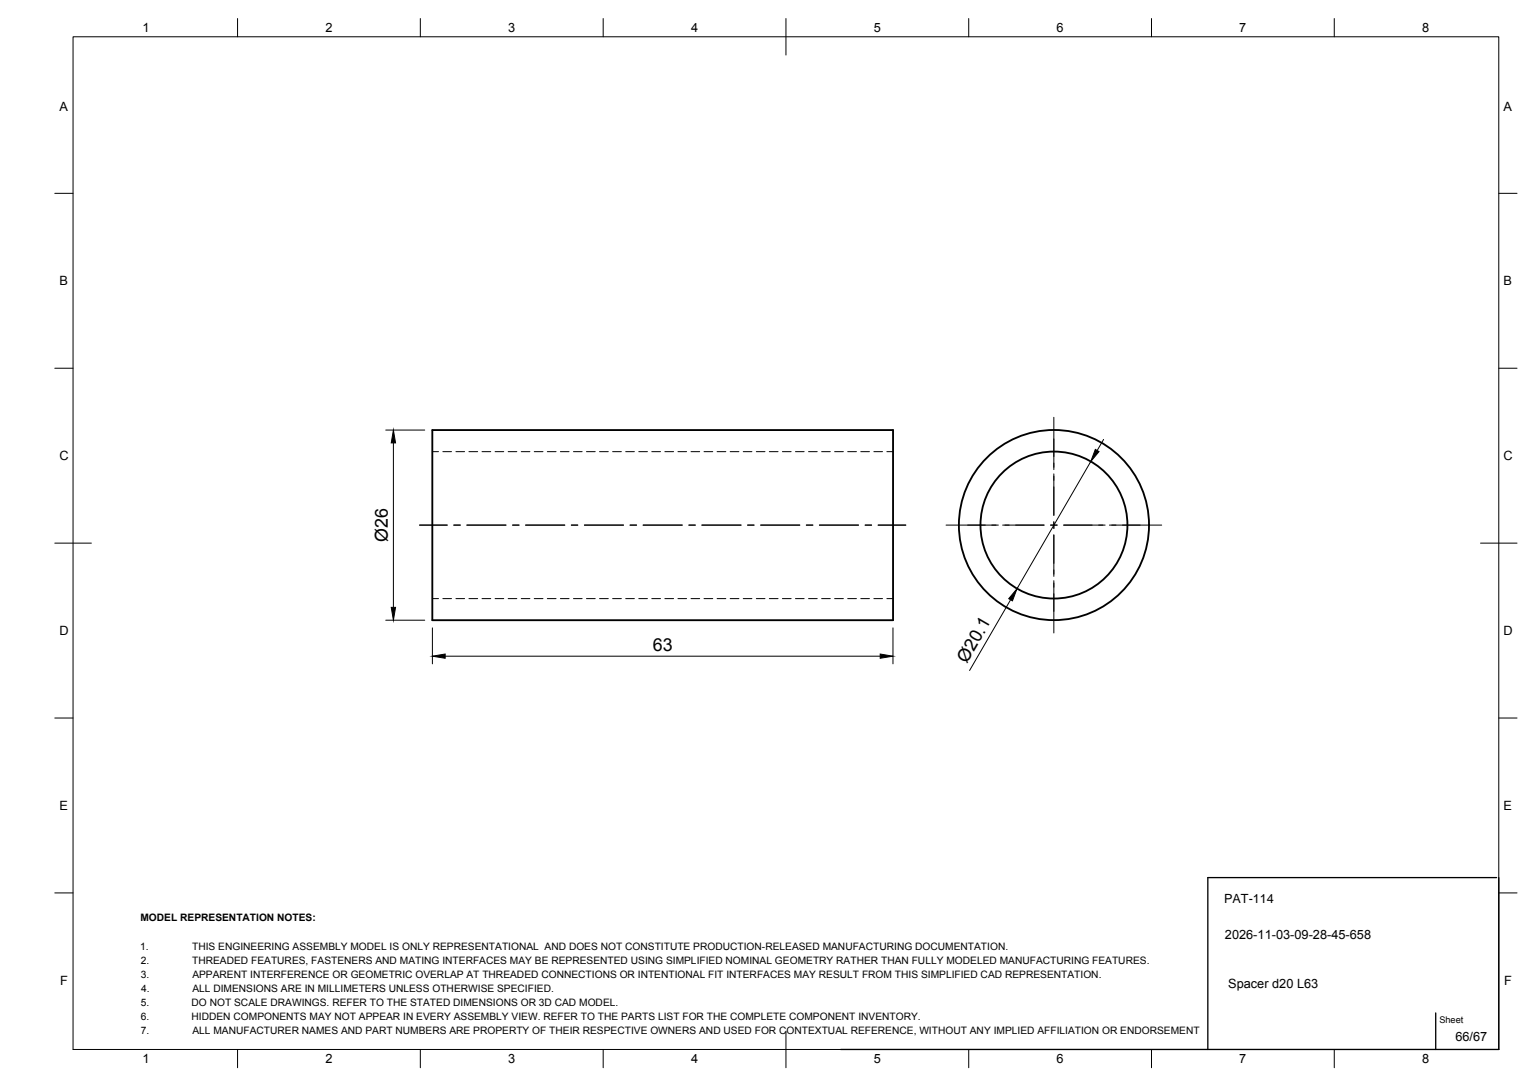
ISO-10303-21;
HEADER;
/* Generated by software containing ST-Developer
 * from STEP Tools, Inc. (www.steptools.com) 
 */

FILE_DESCRIPTION(
/* description */ ('Two-stage gear reducer in split housing'),
/* implementation_level */ '2;1');

FILE_NAME(
/* name */ 'Spacer d20 L63.step',
/* time_stamp */ '2026-10-28T03:22:31-07:00',
/* author */ (''),
/* organization */ (''),
/* preprocessor_version */ 'ST-DEVELOPER v20.2',
/* originating_system */ 'Autodesk Translation Framework v15.17.0.0',
/* authorisation */ '');

FILE_SCHEMA (('AUTOMOTIVE_DESIGN { 1 0 10303 214 3 1 1 }'));
ENDSEC;

DATA;
#10=MECHANICAL_DESIGN_GEOMETRIC_PRESENTATION_REPRESENTATION('',(#1300),#73366);
#1173=SHAPE_REPRESENTATION_RELATIONSHIP('SRR','None',#73665,#1229);
#1229=ADVANCED_BREP_SHAPE_REPRESENTATION('',(#1369),#73361);
#1300=STYLED_ITEM('',(#73981),#1369);
#1369=MANIFOLD_SOLID_BREP('Body1',#16190);
#1594=FACE_BOUND('',#3853,.T.);
#1595=FACE_BOUND('',#3855,.T.);
#1933=PLANE('',#18206);
#1934=PLANE('',#18207);
#2717=FACE_OUTER_BOUND('',#3850,.T.);
#2718=FACE_OUTER_BOUND('',#3851,.T.);
#2719=FACE_OUTER_BOUND('',#3852,.T.);
#2720=FACE_OUTER_BOUND('',#3854,.T.);
#3850=EDGE_LOOP('',(#13795,#13796,#13797,#13798));
#3851=EDGE_LOOP('',(#13799,#13800,#13801,#13802));
#3852=EDGE_LOOP('',(#13803));
#3853=EDGE_LOOP('',(#13804));
#3854=EDGE_LOOP('',(#13805));
#3855=EDGE_LOOP('',(#13806));
#4860=LINE('',#49515,#5884);
#4861=LINE('',#49521,#5885);
#5884=VECTOR('',#22042,1.005);
#5885=VECTOR('',#22049,1.3);
#6728=CIRCLE('',#18201,1.005);
#6729=CIRCLE('',#18202,1.005);
#6730=CIRCLE('',#18204,1.3);
#6731=CIRCLE('',#18205,1.3);
#7937=VERTEX_POINT('',#49512);
#7938=VERTEX_POINT('',#49514);
#7939=VERTEX_POINT('',#49518);
#7940=VERTEX_POINT('',#49520);
#9951=EDGE_CURVE('',#7937,#7937,#6728,.T.);
#9952=EDGE_CURVE('',#7937,#7938,#4860,.T.);
#9953=EDGE_CURVE('',#7938,#7938,#6729,.T.);
#9954=EDGE_CURVE('',#7939,#7939,#6730,.T.);
#9955=EDGE_CURVE('',#7939,#7940,#4861,.T.);
#9956=EDGE_CURVE('',#7940,#7940,#6731,.T.);
#13795=ORIENTED_EDGE('',*,*,#9951,.F.);
#13796=ORIENTED_EDGE('',*,*,#9952,.T.);
#13797=ORIENTED_EDGE('',*,*,#9953,.T.);
#13798=ORIENTED_EDGE('',*,*,#9952,.F.);
#13799=ORIENTED_EDGE('',*,*,#9954,.F.);
#13800=ORIENTED_EDGE('',*,*,#9955,.T.);
#13801=ORIENTED_EDGE('',*,*,#9956,.T.);
#13802=ORIENTED_EDGE('',*,*,#9955,.F.);
#13803=ORIENTED_EDGE('',*,*,#9954,.T.);
#13804=ORIENTED_EDGE('',*,*,#9951,.T.);
#13805=ORIENTED_EDGE('',*,*,#9956,.F.);
#13806=ORIENTED_EDGE('',*,*,#9953,.F.);
#15162=CYLINDRICAL_SURFACE('',#18200,1.005);
#15163=CYLINDRICAL_SURFACE('',#18203,1.3);
#15924=ADVANCED_FACE('',(#2717),#15162,.F.);
#15925=ADVANCED_FACE('',(#2718),#15163,.T.);
#15926=ADVANCED_FACE('',(#2719,#1594),#1933,.T.);
#15927=ADVANCED_FACE('',(#2720,#1595),#1934,.F.);
#16190=CLOSED_SHELL('',(#15924,#15925,#15926,#15927));
#18199=AXIS2_PLACEMENT_3D('',#49510,#22036,#22037);
#18200=AXIS2_PLACEMENT_3D('',#49511,#22038,#22039);
#18201=AXIS2_PLACEMENT_3D('',#49513,#22040,#22041);
#18202=AXIS2_PLACEMENT_3D('',#49516,#22043,#22044);
#18203=AXIS2_PLACEMENT_3D('',#49517,#22045,#22046);
#18204=AXIS2_PLACEMENT_3D('',#49519,#22047,#22048);
#18205=AXIS2_PLACEMENT_3D('',#49522,#22050,#22051);
#18206=AXIS2_PLACEMENT_3D('',#49523,#22052,#22053);
#18207=AXIS2_PLACEMENT_3D('',#49524,#22054,#22055);
#22036=DIRECTION('axis',(0.,0.,1.));
#22037=DIRECTION('refdir',(1.,0.,0.));
#22038=DIRECTION('center_axis',(0.,1.,0.));
#22039=DIRECTION('ref_axis',(1.,0.,0.));
#22040=DIRECTION('center_axis',(0.,-1.,0.));
#22041=DIRECTION('ref_axis',(1.,0.,0.));
#22042=DIRECTION('',(0.,-1.,0.));
#22043=DIRECTION('center_axis',(0.,-1.,0.));
#22044=DIRECTION('ref_axis',(1.,0.,0.));
#22045=DIRECTION('center_axis',(0.,1.,0.));
#22046=DIRECTION('ref_axis',(1.,0.,0.));
#22047=DIRECTION('center_axis',(0.,1.,0.));
#22048=DIRECTION('ref_axis',(1.,0.,0.));
#22049=DIRECTION('',(0.,-1.,0.));
#22050=DIRECTION('center_axis',(0.,1.,0.));
#22051=DIRECTION('ref_axis',(1.,0.,0.));
#22052=DIRECTION('center_axis',(0.,1.,0.));
#22053=DIRECTION('ref_axis',(1.,0.,0.));
#22054=DIRECTION('center_axis',(0.,1.,0.));
#22055=DIRECTION('ref_axis',(1.,0.,0.));
#49510=CARTESIAN_POINT('',(0.,0.,0.));
#49511=CARTESIAN_POINT('Origin',(12.,-5.3,10.));
#49512=CARTESIAN_POINT('',(10.995,1.,10.));
#49513=CARTESIAN_POINT('Origin',(12.,1.,10.));
#49514=CARTESIAN_POINT('',(10.995,-5.3,10.));
#49515=CARTESIAN_POINT('',(10.995,-5.3,10.));
#49516=CARTESIAN_POINT('Origin',(12.,-5.3,10.));
#49517=CARTESIAN_POINT('Origin',(12.,-5.3,10.));
#49518=CARTESIAN_POINT('',(10.7,1.,10.));
#49519=CARTESIAN_POINT('Origin',(12.,1.,10.));
#49520=CARTESIAN_POINT('',(10.7,-5.3,10.));
#49521=CARTESIAN_POINT('',(10.7,-5.3,10.));
#49522=CARTESIAN_POINT('Origin',(12.,-5.3,10.));
#49523=CARTESIAN_POINT('Origin',(12.,1.,10.));
#49524=CARTESIAN_POINT('Origin',(12.,-5.3,10.));
#73297=UNCERTAINTY_MEASURE_WITH_UNIT(LENGTH_MEASURE(0.001),#73367,
'DISTANCE_ACCURACY_VALUE',
'Maximum model space distance between geometric entities at asserted c
onnectivities');
#73302=UNCERTAINTY_MEASURE_WITH_UNIT(LENGTH_MEASURE(0.001),#73367,
'DISTANCE_ACCURACY_VALUE',
'Maximum model space distance between geometric entities at asserted c
onnectivities');
#73361=(
GEOMETRIC_REPRESENTATION_CONTEXT(3)
GLOBAL_UNCERTAINTY_ASSIGNED_CONTEXT((#73297))
GLOBAL_UNIT_ASSIGNED_CONTEXT((#73367,#73369,#73370))
REPRESENTATION_CONTEXT('','3D')
);
#73366=(
GEOMETRIC_REPRESENTATION_CONTEXT(3)
GLOBAL_UNCERTAINTY_ASSIGNED_CONTEXT((#73302))
GLOBAL_UNIT_ASSIGNED_CONTEXT((#73367,#73369,#73370))
REPRESENTATION_CONTEXT('','3D')
);
#73367=(
LENGTH_UNIT()
NAMED_UNIT(*)
SI_UNIT(.CENTI.,.METRE.)
);
#73369=(
NAMED_UNIT(*)
PLANE_ANGLE_UNIT()
SI_UNIT($,.RADIAN.)
);
#73370=(
NAMED_UNIT(*)
SI_UNIT($,.STERADIAN.)
SOLID_ANGLE_UNIT()
);
#73429=SHAPE_DEFINITION_REPRESENTATION(#73562,#73665);
#73562=PRODUCT_DEFINITION_SHAPE('',$,#73729);
#73665=SHAPE_REPRESENTATION('',(#18199),#73361);
#73670=PRODUCT_DEFINITION_CONTEXT('part definition',#73861,'design');
#73729=PRODUCT_DEFINITION('Spacer d20 L63','Spacer d20 L63',#73792,#73670);
#73792=PRODUCT_DEFINITION_FORMATION('',$,#73921);
#73861=APPLICATION_CONTEXT(
'Core Data for Automotive Mechanical Design Process');
#73862=PRODUCT_CONTEXT('part definition',#73861,'mechanical');
#73921=PRODUCT('Spacer d20 L63','Spacer d20 L63','Spacer d20 L63',(#73862));
#73975=COLOUR_RGB('Sky Blue',0.24,0.69,0.87);
#73976=FILL_AREA_STYLE_COLOUR('',#73975);
#73977=FILL_AREA_STYLE('',(#73976));
#73978=SURFACE_STYLE_FILL_AREA(#73977);
#73979=SURFACE_SIDE_STYLE('',(#73978));
#73980=SURFACE_STYLE_USAGE(.BOTH.,#73979);
#73981=PRESENTATION_STYLE_ASSIGNMENT((#73980));
ENDSEC;
END-ISO-10303-21;
